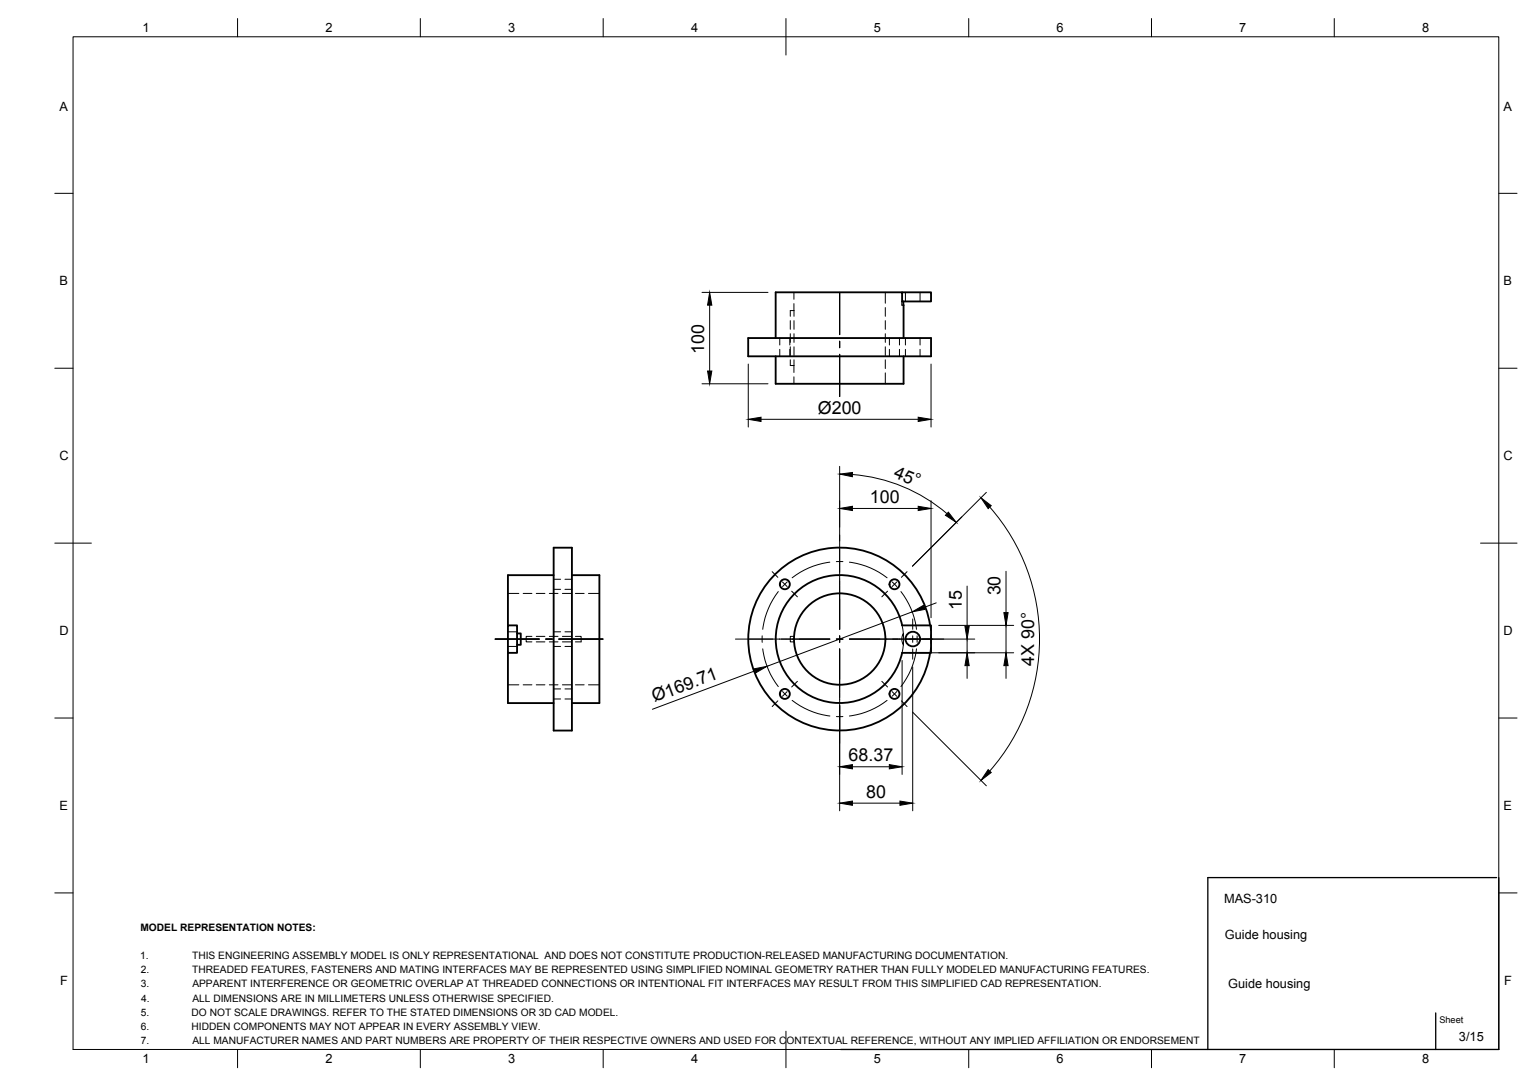
ISO-10303-21;
HEADER;
/* Generated by software containing ST-Developer
 * from STEP Tools, Inc. (www.steptools.com) 
 */

FILE_DESCRIPTION(
/* description */ ('Independent30mm screw-fed quill/spindle unit with16mm straight tool s
ocket, radial set screw, native reusable open ball bearings, retained 
inner/outer race stacks, keyed quill guide and M12x1.75 fine feed. Ext
ernal moving drive and tool not included. Ideal cage orbital links; in
dividual ball spin, force and preload not simulated. No drilling capac
ity, runout, speed, torque, load, life or machine safety rating.'),
/* implementation_level */ '2;1');

FILE_NAME(
/* name */ 'Guide housing.step',
/* time_stamp */ '2026-11-08T18:59:42-08:00',
/* author */ (''),
/* organization */ (''),
/* preprocessor_version */ 'ST-DEVELOPER v20.2',
/* originating_system */ 'Autodesk Translation Framework v15.17.0.0',
/* authorisation */ '');

FILE_SCHEMA (('AUTOMOTIVE_DESIGN { 1 0 10303 214 3 1 1 }'));
ENDSEC;

DATA;
#10=MECHANICAL_DESIGN_GEOMETRIC_PRESENTATION_REPRESENTATION('',(#1592),#63898);
#1556=SHAPE_REPRESENTATION_RELATIONSHIP('SRR','None',#63995,#1574);
#1574=ADVANCED_BREP_SHAPE_REPRESENTATION('',(#1610),#63880);
#1592=STYLED_ITEM('',(#64094),#1610);
#1610=MANIFOLD_SOLID_BREP('Body1',#15478);
#1628=FACE_BOUND('',#3516,.T.);
#1629=FACE_BOUND('',#3518,.T.);
#1630=FACE_BOUND('',#3519,.T.);
#1631=FACE_BOUND('',#3520,.T.);
#1632=FACE_BOUND('',#3521,.T.);
#1633=FACE_BOUND('',#3522,.T.);
#1634=FACE_BOUND('',#3523,.T.);
#1635=FACE_BOUND('',#3525,.T.);
#1636=FACE_BOUND('',#3526,.T.);
#1637=FACE_BOUND('',#3527,.T.);
#1638=FACE_BOUND('',#3528,.T.);
#1639=FACE_BOUND('',#3529,.T.);
#1640=FACE_BOUND('',#3530,.T.);
#1641=FACE_BOUND('',#3535,.T.);
#1642=FACE_BOUND('',#3536,.T.);
#1643=FACE_BOUND('',#3538,.T.);
#1715=CYLINDRICAL_SURFACE('',#15709,12.);
#1716=CYLINDRICAL_SURFACE('',#15711,70.);
#1717=CYLINDRICAL_SURFACE('',#15717,8.);
#1718=CYLINDRICAL_SURFACE('',#15720,8.);
#1719=CYLINDRICAL_SURFACE('',#15723,5.5);
#1720=CYLINDRICAL_SURFACE('',#15726,5.5);
#1721=CYLINDRICAL_SURFACE('',#15729,5.5);
#1722=CYLINDRICAL_SURFACE('',#15732,5.5);
#1723=CYLINDRICAL_SURFACE('',#15744,100.);
#1724=CYLINDRICAL_SURFACE('',#15745,70.);
#1725=CYLINDRICAL_SURFACE('',#15747,50.);
#2380=CIRCLE('',#15699,50.);
#2381=CIRCLE('',#15700,50.);
#2382=CIRCLE('',#15704,50.);
#2383=CIRCLE('',#15705,50.);
#2384=CIRCLE('',#15707,70.);
#2385=CIRCLE('',#15708,12.);
#2386=CIRCLE('',#15710,12.);
#2387=CIRCLE('',#15712,70.);
#2388=CIRCLE('',#15713,70.);
#2389=CIRCLE('',#15714,70.);
#2390=CIRCLE('',#15715,70.);
#2391=CIRCLE('',#15716,70.);
#2392=CIRCLE('',#15718,8.);
#2393=CIRCLE('',#15719,8.);
#2394=CIRCLE('',#15721,8.);
#2395=CIRCLE('',#15722,8.);
#2396=CIRCLE('',#15724,5.5);
#2397=CIRCLE('',#15725,5.5);
#2398=CIRCLE('',#15727,5.5);
#2399=CIRCLE('',#15728,5.5);
#2400=CIRCLE('',#15730,5.5);
#2401=CIRCLE('',#15731,5.5);
#2402=CIRCLE('',#15733,5.5);
#2403=CIRCLE('',#15734,5.5);
#2404=CIRCLE('',#15740,100.);
#2405=CIRCLE('',#15742,100.);
#2406=CIRCLE('',#15743,70.);
#2407=CIRCLE('',#15746,70.);
#2408=CIRCLE('',#15748,50.);
#2409=CIRCLE('',#15749,50.);
#2660=FACE_OUTER_BOUND('',#3498,.T.);
#2661=FACE_OUTER_BOUND('',#3499,.T.);
#2662=FACE_OUTER_BOUND('',#3500,.T.);
#2663=FACE_OUTER_BOUND('',#3501,.T.);
#2664=FACE_OUTER_BOUND('',#3502,.T.);
#2665=FACE_OUTER_BOUND('',#3503,.T.);
#2666=FACE_OUTER_BOUND('',#3504,.T.);
#2667=FACE_OUTER_BOUND('',#3505,.T.);
#2668=FACE_OUTER_BOUND('',#3506,.T.);
#2669=FACE_OUTER_BOUND('',#3507,.T.);
#2670=FACE_OUTER_BOUND('',#3508,.T.);
#2671=FACE_OUTER_BOUND('',#3509,.T.);
#2672=FACE_OUTER_BOUND('',#3510,.T.);
#2673=FACE_OUTER_BOUND('',#3511,.T.);
#2674=FACE_OUTER_BOUND('',#3512,.T.);
#2675=FACE_OUTER_BOUND('',#3513,.T.);
#2676=FACE_OUTER_BOUND('',#3514,.T.);
#2677=FACE_OUTER_BOUND('',#3515,.T.);
#2678=FACE_OUTER_BOUND('',#3517,.T.);
#2679=FACE_OUTER_BOUND('',#3524,.T.);
#2680=FACE_OUTER_BOUND('',#3531,.T.);
#2681=FACE_OUTER_BOUND('',#3532,.T.);
#2682=FACE_OUTER_BOUND('',#3533,.T.);
#2683=FACE_OUTER_BOUND('',#3534,.T.);
#2684=FACE_OUTER_BOUND('',#3537,.T.);
#3498=EDGE_LOOP('',(#9844,#9845,#9846,#9847));
#3499=EDGE_LOOP('',(#9848,#9849,#9850,#9851,#9852));
#3500=EDGE_LOOP('',(#9853,#9854,#9855,#9856));
#3501=EDGE_LOOP('',(#9857,#9858,#9859,#9860));
#3502=EDGE_LOOP('',(#9861,#9862,#9863,#9864,#9865));
#3503=EDGE_LOOP('',(#9866,#9867));
#3504=EDGE_LOOP('',(#9868,#9869,#9870,#9871));
#3505=EDGE_LOOP('',(#9872,#9873,#9874,#9875,#9876,#9877,#9878,#9879,#9880,
#9881,#9882,#9883));
#3506=EDGE_LOOP('',(#9884,#9885,#9886,#9887));
#3507=EDGE_LOOP('',(#9888,#9889,#9890,#9891));
#3508=EDGE_LOOP('',(#9892,#9893,#9894,#9895));
#3509=EDGE_LOOP('',(#9896,#9897,#9898,#9899));
#3510=EDGE_LOOP('',(#9900,#9901,#9902,#9903));
#3511=EDGE_LOOP('',(#9904,#9905,#9906,#9907));
#3512=EDGE_LOOP('',(#9908,#9909,#9910,#9911));
#3513=EDGE_LOOP('',(#9912,#9913,#9914,#9915));
#3514=EDGE_LOOP('',(#9916,#9917,#9918,#9919));
#3515=EDGE_LOOP('',(#9920,#9921,#9922,#9923,#9924,#9925));
#3516=EDGE_LOOP('',(#9926));
#3517=EDGE_LOOP('',(#9927));
#3518=EDGE_LOOP('',(#9928));
#3519=EDGE_LOOP('',(#9929));
#3520=EDGE_LOOP('',(#9930));
#3521=EDGE_LOOP('',(#9931));
#3522=EDGE_LOOP('',(#9932));
#3523=EDGE_LOOP('',(#9933));
#3524=EDGE_LOOP('',(#9934));
#3525=EDGE_LOOP('',(#9935));
#3526=EDGE_LOOP('',(#9936));
#3527=EDGE_LOOP('',(#9937));
#3528=EDGE_LOOP('',(#9938));
#3529=EDGE_LOOP('',(#9939));
#3530=EDGE_LOOP('',(#9940));
#3531=EDGE_LOOP('',(#9941,#9942,#9943,#9944));
#3532=EDGE_LOOP('',(#9945,#9946,#9947,#9948));
#3533=EDGE_LOOP('',(#9949,#9950,#9951,#9952,#9953,#9954,#9955,#9956,#9957,
#9958,#9959,#9960));
#3534=EDGE_LOOP('',(#9961,#9962,#9963,#9964,#9965));
#3535=EDGE_LOOP('',(#9966));
#3536=EDGE_LOOP('',(#9967));
#3537=EDGE_LOOP('',(#9968));
#3538=EDGE_LOOP('',(#9969));
#4423=LINE('',#19955,#5186);
#4424=LINE('',#19957,#5187);
#4425=LINE('',#19959,#5188);
#4426=LINE('',#19960,#5189);
#4427=LINE('',#19965,#5190);
#4428=LINE('',#19967,#5191);
#4429=LINE('',#19971,#5192);
#4430=LINE('',#19973,#5193);
#4431=LINE('',#19974,#5194);
#4432=LINE('',#19976,#5195);
#4433=LINE('',#19988,#5196);
#4434=LINE('',#19991,#5197);
#4435=LINE('',#19996,#5198);
#4436=LINE('',#20000,#5199);
#4437=LINE('',#20005,#5200);
#4438=LINE('',#20011,#5201);
#4439=LINE('',#20017,#5202);
#4440=LINE('',#20023,#5203);
#4441=LINE('',#20029,#5204);
#4442=LINE('',#20035,#5205);
#4443=LINE('',#20041,#5206);
#4444=LINE('',#20045,#5207);
#4445=LINE('',#20047,#5208);
#4446=LINE('',#20048,#5209);
#4447=LINE('',#20051,#5210);
#4448=LINE('',#20053,#5211);
#4449=LINE('',#20054,#5212);
#4450=LINE('',#20056,#5213);
#4451=LINE('',#20057,#5214);
#4452=LINE('',#20068,#5215);
#4453=LINE('',#20071,#5216);
#4454=LINE('',#20076,#5217);
#4455=LINE('',#20078,#5218);
#5186=VECTOR('',#16865,10.);
#5187=VECTOR('',#16866,10.);
#5188=VECTOR('',#16867,10.);
#5189=VECTOR('',#16868,10.);
#5190=VECTOR('',#16873,10.);
#5191=VECTOR('',#16874,10.);
#5192=VECTOR('',#16879,10.);
#5193=VECTOR('',#16880,10.);
#5194=VECTOR('',#16881,10.);
#5195=VECTOR('',#16884,10.);
#5196=VECTOR('',#16899,10.);
#5197=VECTOR('',#16902,10.);
#5198=VECTOR('',#16907,10.);
#5199=VECTOR('',#16910,70.);
#5200=VECTOR('',#16915,10.);
#5201=VECTOR('',#16922,8.);
#5202=VECTOR('',#16929,8.);
#5203=VECTOR('',#16936,5.5);
#5204=VECTOR('',#16943,5.5);
#5205=VECTOR('',#16950,5.5);
#5206=VECTOR('',#16957,5.5);
#5207=VECTOR('',#16962,10.);
#5208=VECTOR('',#16963,10.);
#5209=VECTOR('',#16964,10.);
#5210=VECTOR('',#16967,10.);
#5211=VECTOR('',#16968,10.);
#5212=VECTOR('',#16969,10.);
#5213=VECTOR('',#16972,10.);
#5214=VECTOR('',#16973,10.);
#5215=VECTOR('',#16988,100.);
#5216=VECTOR('',#16991,70.);
#5217=VECTOR('',#16998,50.);
#5218=VECTOR('',#16999,50.);
#5949=VERTEX_POINT('',#19953);
#5950=VERTEX_POINT('',#19954);
#5951=VERTEX_POINT('',#19956);
#5952=VERTEX_POINT('',#19958);
#5953=VERTEX_POINT('',#19962);
#5954=VERTEX_POINT('',#19964);
#5955=VERTEX_POINT('',#19966);
#5956=VERTEX_POINT('',#19970);
#5957=VERTEX_POINT('',#19972);
#5958=VERTEX_POINT('',#19978);
#5959=VERTEX_POINT('',#19982);
#5960=VERTEX_POINT('',#19983);
#5961=VERTEX_POINT('',#19987);
#5962=VERTEX_POINT('',#19989);
#5963=VERTEX_POINT('',#19993);
#5964=VERTEX_POINT('',#19995);
#5965=VERTEX_POINT('',#19997);
#5966=VERTEX_POINT('',#19999);
#5967=VERTEX_POINT('',#20002);
#5968=VERTEX_POINT('',#20004);
#5969=VERTEX_POINT('',#20008);
#5970=VERTEX_POINT('',#20010);
#5971=VERTEX_POINT('',#20014);
#5972=VERTEX_POINT('',#20016);
#5973=VERTEX_POINT('',#20020);
#5974=VERTEX_POINT('',#20022);
#5975=VERTEX_POINT('',#20026);
#5976=VERTEX_POINT('',#20028);
#5977=VERTEX_POINT('',#20032);
#5978=VERTEX_POINT('',#20034);
#5979=VERTEX_POINT('',#20038);
#5980=VERTEX_POINT('',#20040);
#5981=VERTEX_POINT('',#20044);
#5982=VERTEX_POINT('',#20046);
#5983=VERTEX_POINT('',#20050);
#5984=VERTEX_POINT('',#20052);
#5985=VERTEX_POINT('',#20060);
#5986=VERTEX_POINT('',#20063);
#5987=VERTEX_POINT('',#20065);
#5988=VERTEX_POINT('',#20070);
#5989=VERTEX_POINT('',#20074);
#5990=VERTEX_POINT('',#20077);
#7511=EDGE_CURVE('',#5949,#5950,#4423,.T.);
#7512=EDGE_CURVE('',#5949,#5951,#4424,.T.);
#7513=EDGE_CURVE('',#5952,#5951,#4425,.T.);
#7514=EDGE_CURVE('',#5952,#5950,#4426,.T.);
#7515=EDGE_CURVE('',#5950,#5953,#2380,.T.);
#7516=EDGE_CURVE('',#5954,#5952,#4427,.T.);
#7517=EDGE_CURVE('',#5955,#5954,#4428,.T.);
#7518=EDGE_CURVE('',#5953,#5955,#2381,.T.);
#7519=EDGE_CURVE('',#5955,#5956,#4429,.T.);
#7520=EDGE_CURVE('',#5954,#5957,#4430,.T.);
#7521=EDGE_CURVE('',#5957,#5956,#4431,.T.);
#7522=EDGE_CURVE('',#5951,#5957,#4432,.T.);
#7523=EDGE_CURVE('',#5956,#5958,#2382,.T.);
#7524=EDGE_CURVE('',#5958,#5949,#2383,.T.);
#7525=EDGE_CURVE('',#5959,#5960,#2384,.T.);
#7526=EDGE_CURVE('',#5960,#5959,#2385,.T.);
#7527=EDGE_CURVE('',#5961,#5959,#4433,.T.);
#7528=EDGE_CURVE('',#5961,#5962,#2386,.T.);
#7529=EDGE_CURVE('',#5960,#5962,#4434,.T.);
#7530=EDGE_CURVE('',#5962,#5963,#2387,.T.);
#7531=EDGE_CURVE('',#5963,#5964,#4435,.T.);
#7532=EDGE_CURVE('',#5965,#5964,#2388,.T.);
#7533=EDGE_CURVE('',#5965,#5966,#4436,.T.);
#7534=EDGE_CURVE('',#5966,#5966,#2389,.T.);
#7535=EDGE_CURVE('',#5967,#5965,#2390,.T.);
#7536=EDGE_CURVE('',#5967,#5968,#4437,.T.);
#7537=EDGE_CURVE('',#5968,#5961,#2391,.T.);
#7538=EDGE_CURVE('',#5969,#5969,#2392,.T.);
#7539=EDGE_CURVE('',#5969,#5970,#4438,.T.);
#7540=EDGE_CURVE('',#5970,#5970,#2393,.T.);
#7541=EDGE_CURVE('',#5971,#5971,#2394,.T.);
#7542=EDGE_CURVE('',#5971,#5972,#4439,.T.);
#7543=EDGE_CURVE('',#5972,#5972,#2395,.T.);
#7544=EDGE_CURVE('',#5973,#5973,#2396,.T.);
#7545=EDGE_CURVE('',#5973,#5974,#4440,.T.);
#7546=EDGE_CURVE('',#5974,#5974,#2397,.T.);
#7547=EDGE_CURVE('',#5975,#5975,#2398,.T.);
#7548=EDGE_CURVE('',#5975,#5976,#4441,.T.);
#7549=EDGE_CURVE('',#5976,#5976,#2399,.T.);
#7550=EDGE_CURVE('',#5977,#5977,#2400,.T.);
#7551=EDGE_CURVE('',#5977,#5978,#4442,.T.);
#7552=EDGE_CURVE('',#5978,#5978,#2401,.T.);
#7553=EDGE_CURVE('',#5979,#5979,#2402,.T.);
#7554=EDGE_CURVE('',#5979,#5980,#4443,.T.);
#7555=EDGE_CURVE('',#5980,#5980,#2403,.T.);
#7556=EDGE_CURVE('',#5981,#5967,#4444,.T.);
#7557=EDGE_CURVE('',#5982,#5981,#4445,.T.);
#7558=EDGE_CURVE('',#5982,#5968,#4446,.T.);
#7559=EDGE_CURVE('',#5983,#5982,#4447,.T.);
#7560=EDGE_CURVE('',#5984,#5981,#4448,.T.);
#7561=EDGE_CURVE('',#5983,#5984,#4449,.T.);
#7562=EDGE_CURVE('',#5963,#5983,#4450,.T.);
#7563=EDGE_CURVE('',#5964,#5984,#4451,.T.);
#7564=EDGE_CURVE('',#5985,#5985,#2404,.T.);
#7565=EDGE_CURVE('',#5986,#5986,#2405,.T.);
#7566=EDGE_CURVE('',#5987,#5987,#2406,.T.);
#7567=EDGE_CURVE('',#5985,#5986,#4452,.T.);
#7568=EDGE_CURVE('',#5987,#5988,#4453,.T.);
#7569=EDGE_CURVE('',#5988,#5988,#2407,.T.);
#7570=EDGE_CURVE('',#5989,#5989,#2408,.T.);
#7571=EDGE_CURVE('',#5989,#5953,#4454,.T.);
#7572=EDGE_CURVE('',#5958,#5990,#4455,.T.);
#7573=EDGE_CURVE('',#5990,#5990,#2409,.T.);
#9844=ORIENTED_EDGE('',*,*,#7511,.F.);
#9845=ORIENTED_EDGE('',*,*,#7512,.T.);
#9846=ORIENTED_EDGE('',*,*,#7513,.F.);
#9847=ORIENTED_EDGE('',*,*,#7514,.T.);
#9848=ORIENTED_EDGE('',*,*,#7515,.F.);
#9849=ORIENTED_EDGE('',*,*,#7514,.F.);
#9850=ORIENTED_EDGE('',*,*,#7516,.F.);
#9851=ORIENTED_EDGE('',*,*,#7517,.F.);
#9852=ORIENTED_EDGE('',*,*,#7518,.F.);
#9853=ORIENTED_EDGE('',*,*,#7519,.F.);
#9854=ORIENTED_EDGE('',*,*,#7517,.T.);
#9855=ORIENTED_EDGE('',*,*,#7520,.T.);
#9856=ORIENTED_EDGE('',*,*,#7521,.T.);
#9857=ORIENTED_EDGE('',*,*,#7516,.T.);
#9858=ORIENTED_EDGE('',*,*,#7513,.T.);
#9859=ORIENTED_EDGE('',*,*,#7522,.T.);
#9860=ORIENTED_EDGE('',*,*,#7520,.F.);
#9861=ORIENTED_EDGE('',*,*,#7523,.F.);
#9862=ORIENTED_EDGE('',*,*,#7521,.F.);
#9863=ORIENTED_EDGE('',*,*,#7522,.F.);
#9864=ORIENTED_EDGE('',*,*,#7512,.F.);
#9865=ORIENTED_EDGE('',*,*,#7524,.F.);
#9866=ORIENTED_EDGE('',*,*,#7525,.F.);
#9867=ORIENTED_EDGE('',*,*,#7526,.F.);
#9868=ORIENTED_EDGE('',*,*,#7527,.F.);
#9869=ORIENTED_EDGE('',*,*,#7528,.T.);
#9870=ORIENTED_EDGE('',*,*,#7529,.F.);
#9871=ORIENTED_EDGE('',*,*,#7526,.T.);
#9872=ORIENTED_EDGE('',*,*,#7527,.T.);
#9873=ORIENTED_EDGE('',*,*,#7525,.T.);
#9874=ORIENTED_EDGE('',*,*,#7529,.T.);
#9875=ORIENTED_EDGE('',*,*,#7530,.T.);
#9876=ORIENTED_EDGE('',*,*,#7531,.T.);
#9877=ORIENTED_EDGE('',*,*,#7532,.F.);
#9878=ORIENTED_EDGE('',*,*,#7533,.T.);
#9879=ORIENTED_EDGE('',*,*,#7534,.T.);
#9880=ORIENTED_EDGE('',*,*,#7533,.F.);
#9881=ORIENTED_EDGE('',*,*,#7535,.F.);
#9882=ORIENTED_EDGE('',*,*,#7536,.T.);
#9883=ORIENTED_EDGE('',*,*,#7537,.T.);
#9884=ORIENTED_EDGE('',*,*,#7538,.F.);
#9885=ORIENTED_EDGE('',*,*,#7539,.T.);
#9886=ORIENTED_EDGE('',*,*,#7540,.F.);
#9887=ORIENTED_EDGE('',*,*,#7539,.F.);
#9888=ORIENTED_EDGE('',*,*,#7541,.F.);
#9889=ORIENTED_EDGE('',*,*,#7542,.T.);
#9890=ORIENTED_EDGE('',*,*,#7543,.F.);
#9891=ORIENTED_EDGE('',*,*,#7542,.F.);
#9892=ORIENTED_EDGE('',*,*,#7544,.F.);
#9893=ORIENTED_EDGE('',*,*,#7545,.T.);
#9894=ORIENTED_EDGE('',*,*,#7546,.F.);
#9895=ORIENTED_EDGE('',*,*,#7545,.F.);
#9896=ORIENTED_EDGE('',*,*,#7547,.F.);
#9897=ORIENTED_EDGE('',*,*,#7548,.T.);
#9898=ORIENTED_EDGE('',*,*,#7549,.F.);
#9899=ORIENTED_EDGE('',*,*,#7548,.F.);
#9900=ORIENTED_EDGE('',*,*,#7550,.F.);
#9901=ORIENTED_EDGE('',*,*,#7551,.T.);
#9902=ORIENTED_EDGE('',*,*,#7552,.F.);
#9903=ORIENTED_EDGE('',*,*,#7551,.F.);
#9904=ORIENTED_EDGE('',*,*,#7553,.F.);
#9905=ORIENTED_EDGE('',*,*,#7554,.T.);
#9906=ORIENTED_EDGE('',*,*,#7555,.F.);
#9907=ORIENTED_EDGE('',*,*,#7554,.F.);
#9908=ORIENTED_EDGE('',*,*,#7536,.F.);
#9909=ORIENTED_EDGE('',*,*,#7556,.F.);
#9910=ORIENTED_EDGE('',*,*,#7557,.F.);
#9911=ORIENTED_EDGE('',*,*,#7558,.T.);
#9912=ORIENTED_EDGE('',*,*,#7559,.T.);
#9913=ORIENTED_EDGE('',*,*,#7557,.T.);
#9914=ORIENTED_EDGE('',*,*,#7560,.F.);
#9915=ORIENTED_EDGE('',*,*,#7561,.F.);
#9916=ORIENTED_EDGE('',*,*,#7531,.F.);
#9917=ORIENTED_EDGE('',*,*,#7562,.T.);
#9918=ORIENTED_EDGE('',*,*,#7561,.T.);
#9919=ORIENTED_EDGE('',*,*,#7563,.F.);
#9920=ORIENTED_EDGE('',*,*,#7537,.F.);
#9921=ORIENTED_EDGE('',*,*,#7558,.F.);
#9922=ORIENTED_EDGE('',*,*,#7559,.F.);
#9923=ORIENTED_EDGE('',*,*,#7562,.F.);
#9924=ORIENTED_EDGE('',*,*,#7530,.F.);
#9925=ORIENTED_EDGE('',*,*,#7528,.F.);
#9926=ORIENTED_EDGE('',*,*,#7540,.T.);
#9927=ORIENTED_EDGE('',*,*,#7564,.T.);
#9928=ORIENTED_EDGE('',*,*,#7541,.T.);
#9929=ORIENTED_EDGE('',*,*,#7534,.F.);
#9930=ORIENTED_EDGE('',*,*,#7553,.T.);
#9931=ORIENTED_EDGE('',*,*,#7550,.T.);
#9932=ORIENTED_EDGE('',*,*,#7547,.T.);
#9933=ORIENTED_EDGE('',*,*,#7544,.T.);
#9934=ORIENTED_EDGE('',*,*,#7565,.F.);
#9935=ORIENTED_EDGE('',*,*,#7543,.T.);
#9936=ORIENTED_EDGE('',*,*,#7566,.F.);
#9937=ORIENTED_EDGE('',*,*,#7555,.T.);
#9938=ORIENTED_EDGE('',*,*,#7552,.T.);
#9939=ORIENTED_EDGE('',*,*,#7549,.T.);
#9940=ORIENTED_EDGE('',*,*,#7546,.T.);
#9941=ORIENTED_EDGE('',*,*,#7564,.F.);
#9942=ORIENTED_EDGE('',*,*,#7567,.T.);
#9943=ORIENTED_EDGE('',*,*,#7565,.T.);
#9944=ORIENTED_EDGE('',*,*,#7567,.F.);
#9945=ORIENTED_EDGE('',*,*,#7566,.T.);
#9946=ORIENTED_EDGE('',*,*,#7568,.T.);
#9947=ORIENTED_EDGE('',*,*,#7569,.T.);
#9948=ORIENTED_EDGE('',*,*,#7568,.F.);
#9949=ORIENTED_EDGE('',*,*,#7570,.F.);
#9950=ORIENTED_EDGE('',*,*,#7571,.T.);
#9951=ORIENTED_EDGE('',*,*,#7518,.T.);
#9952=ORIENTED_EDGE('',*,*,#7519,.T.);
#9953=ORIENTED_EDGE('',*,*,#7523,.T.);
#9954=ORIENTED_EDGE('',*,*,#7572,.T.);
#9955=ORIENTED_EDGE('',*,*,#7573,.T.);
#9956=ORIENTED_EDGE('',*,*,#7572,.F.);
#9957=ORIENTED_EDGE('',*,*,#7524,.T.);
#9958=ORIENTED_EDGE('',*,*,#7511,.T.);
#9959=ORIENTED_EDGE('',*,*,#7515,.T.);
#9960=ORIENTED_EDGE('',*,*,#7571,.F.);
#9961=ORIENTED_EDGE('',*,*,#7535,.T.);
#9962=ORIENTED_EDGE('',*,*,#7532,.T.);
#9963=ORIENTED_EDGE('',*,*,#7563,.T.);
#9964=ORIENTED_EDGE('',*,*,#7560,.T.);
#9965=ORIENTED_EDGE('',*,*,#7556,.T.);
#9966=ORIENTED_EDGE('',*,*,#7538,.T.);
#9967=ORIENTED_EDGE('',*,*,#7570,.T.);
#9968=ORIENTED_EDGE('',*,*,#7569,.F.);
#9969=ORIENTED_EDGE('',*,*,#7573,.F.);
#14510=PLANE('',#15697);
#14511=PLANE('',#15698);
#14512=PLANE('',#15701);
#14513=PLANE('',#15702);
#14514=PLANE('',#15703);
#14515=PLANE('',#15706);
#14516=PLANE('',#15735);
#14517=PLANE('',#15736);
#14518=PLANE('',#15737);
#14519=PLANE('',#15738);
#14520=PLANE('',#15739);
#14521=PLANE('',#15741);
#14522=PLANE('',#15750);
#14523=PLANE('',#15751);
#14640=ADVANCED_FACE('',(#2660),#14510,.F.);
#14641=ADVANCED_FACE('',(#2661),#14511,.F.);
#14642=ADVANCED_FACE('',(#2662),#14512,.F.);
#14643=ADVANCED_FACE('',(#2663),#14513,.F.);
#14644=ADVANCED_FACE('',(#2664),#14514,.F.);
#14645=ADVANCED_FACE('',(#2665),#14515,.F.);
#14646=ADVANCED_FACE('',(#2666),#1715,.F.);
#14647=ADVANCED_FACE('',(#2667),#1716,.T.);
#14648=ADVANCED_FACE('',(#2668),#1717,.F.);
#14649=ADVANCED_FACE('',(#2669),#1718,.F.);
#14650=ADVANCED_FACE('',(#2670),#1719,.F.);
#14651=ADVANCED_FACE('',(#2671),#1720,.F.);
#14652=ADVANCED_FACE('',(#2672),#1721,.F.);
#14653=ADVANCED_FACE('',(#2673),#1722,.F.);
#14654=ADVANCED_FACE('',(#2674),#14516,.T.);
#14655=ADVANCED_FACE('',(#2675),#14517,.T.);
#14656=ADVANCED_FACE('',(#2676),#14518,.T.);
#14657=ADVANCED_FACE('',(#2677,#1628),#14519,.F.);
#14658=ADVANCED_FACE('',(#2678,#1629,#1630,#1631,#1632,#1633,#1634),#14520,
 .T.);
#14659=ADVANCED_FACE('',(#2679,#1635,#1636,#1637,#1638,#1639,#1640),#14521,
 .F.);
#14660=ADVANCED_FACE('',(#2680),#1723,.T.);
#14661=ADVANCED_FACE('',(#2681),#1724,.T.);
#14662=ADVANCED_FACE('',(#2682),#1725,.F.);
#14663=ADVANCED_FACE('',(#2683,#1641,#1642),#14522,.T.);
#14664=ADVANCED_FACE('',(#2684,#1643),#14523,.F.);
#15478=CLOSED_SHELL('',(#14640,#14641,#14642,#14643,#14644,#14645,#14646,
#14647,#14648,#14649,#14650,#14651,#14652,#14653,#14654,#14655,#14656,#14657,
#14658,#14659,#14660,#14661,#14662,#14663,#14664));
#15696=AXIS2_PLACEMENT_3D('',#19951,#16861,#16862);
#15697=AXIS2_PLACEMENT_3D('',#19952,#16863,#16864);
#15698=AXIS2_PLACEMENT_3D('',#19961,#16869,#16870);
#15699=AXIS2_PLACEMENT_3D('',#19963,#16871,#16872);
#15700=AXIS2_PLACEMENT_3D('',#19968,#16875,#16876);
#15701=AXIS2_PLACEMENT_3D('',#19969,#16877,#16878);
#15702=AXIS2_PLACEMENT_3D('',#19975,#16882,#16883);
#15703=AXIS2_PLACEMENT_3D('',#19977,#16885,#16886);
#15704=AXIS2_PLACEMENT_3D('',#19979,#16887,#16888);
#15705=AXIS2_PLACEMENT_3D('',#19980,#16889,#16890);
#15706=AXIS2_PLACEMENT_3D('',#19981,#16891,#16892);
#15707=AXIS2_PLACEMENT_3D('',#19984,#16893,#16894);
#15708=AXIS2_PLACEMENT_3D('',#19985,#16895,#16896);
#15709=AXIS2_PLACEMENT_3D('',#19986,#16897,#16898);
#15710=AXIS2_PLACEMENT_3D('',#19990,#16900,#16901);
#15711=AXIS2_PLACEMENT_3D('',#19992,#16903,#16904);
#15712=AXIS2_PLACEMENT_3D('',#19994,#16905,#16906);
#15713=AXIS2_PLACEMENT_3D('',#19998,#16908,#16909);
#15714=AXIS2_PLACEMENT_3D('',#20001,#16911,#16912);
#15715=AXIS2_PLACEMENT_3D('',#20003,#16913,#16914);
#15716=AXIS2_PLACEMENT_3D('',#20006,#16916,#16917);
#15717=AXIS2_PLACEMENT_3D('',#20007,#16918,#16919);
#15718=AXIS2_PLACEMENT_3D('',#20009,#16920,#16921);
#15719=AXIS2_PLACEMENT_3D('',#20012,#16923,#16924);
#15720=AXIS2_PLACEMENT_3D('',#20013,#16925,#16926);
#15721=AXIS2_PLACEMENT_3D('',#20015,#16927,#16928);
#15722=AXIS2_PLACEMENT_3D('',#20018,#16930,#16931);
#15723=AXIS2_PLACEMENT_3D('',#20019,#16932,#16933);
#15724=AXIS2_PLACEMENT_3D('',#20021,#16934,#16935);
#15725=AXIS2_PLACEMENT_3D('',#20024,#16937,#16938);
#15726=AXIS2_PLACEMENT_3D('',#20025,#16939,#16940);
#15727=AXIS2_PLACEMENT_3D('',#20027,#16941,#16942);
#15728=AXIS2_PLACEMENT_3D('',#20030,#16944,#16945);
#15729=AXIS2_PLACEMENT_3D('',#20031,#16946,#16947);
#15730=AXIS2_PLACEMENT_3D('',#20033,#16948,#16949);
#15731=AXIS2_PLACEMENT_3D('',#20036,#16951,#16952);
#15732=AXIS2_PLACEMENT_3D('',#20037,#16953,#16954);
#15733=AXIS2_PLACEMENT_3D('',#20039,#16955,#16956);
#15734=AXIS2_PLACEMENT_3D('',#20042,#16958,#16959);
#15735=AXIS2_PLACEMENT_3D('',#20043,#16960,#16961);
#15736=AXIS2_PLACEMENT_3D('',#20049,#16965,#16966);
#15737=AXIS2_PLACEMENT_3D('',#20055,#16970,#16971);
#15738=AXIS2_PLACEMENT_3D('',#20058,#16974,#16975);
#15739=AXIS2_PLACEMENT_3D('',#20059,#16976,#16977);
#15740=AXIS2_PLACEMENT_3D('',#20061,#16978,#16979);
#15741=AXIS2_PLACEMENT_3D('',#20062,#16980,#16981);
#15742=AXIS2_PLACEMENT_3D('',#20064,#16982,#16983);
#15743=AXIS2_PLACEMENT_3D('',#20066,#16984,#16985);
#15744=AXIS2_PLACEMENT_3D('',#20067,#16986,#16987);
#15745=AXIS2_PLACEMENT_3D('',#20069,#16989,#16990);
#15746=AXIS2_PLACEMENT_3D('',#20072,#16992,#16993);
#15747=AXIS2_PLACEMENT_3D('',#20073,#16994,#16995);
#15748=AXIS2_PLACEMENT_3D('',#20075,#16996,#16997);
#15749=AXIS2_PLACEMENT_3D('',#20079,#17000,#17001);
#15750=AXIS2_PLACEMENT_3D('',#20080,#17002,#17003);
#15751=AXIS2_PLACEMENT_3D('',#20081,#17004,#17005);
#16861=DIRECTION('axis',(0.,0.,1.));
#16862=DIRECTION('refdir',(1.,0.,0.));
#16863=DIRECTION('center_axis',(0.,-1.,0.));
#16864=DIRECTION('ref_axis',(-1.,0.,0.));
#16865=DIRECTION('',(0.,0.,1.));
#16866=DIRECTION('',(-1.,0.,0.));
#16867=DIRECTION('',(0.,0.,-1.));
#16868=DIRECTION('',(1.,0.,0.));
#16869=DIRECTION('center_axis',(0.,0.,1.));
#16870=DIRECTION('ref_axis',(1.,0.,0.));
#16871=DIRECTION('center_axis',(0.,0.,-1.));
#16872=DIRECTION('ref_axis',(1.,0.,0.));
#16873=DIRECTION('',(0.,-1.,0.));
#16874=DIRECTION('',(-1.,0.,0.));
#16875=DIRECTION('center_axis',(0.,0.,-1.));
#16876=DIRECTION('ref_axis',(1.,0.,0.));
#16877=DIRECTION('center_axis',(0.,1.,0.));
#16878=DIRECTION('ref_axis',(1.,0.,0.));
#16879=DIRECTION('',(0.,0.,-1.));
#16880=DIRECTION('',(0.,0.,-1.));
#16881=DIRECTION('',(1.,0.,0.));
#16882=DIRECTION('center_axis',(-1.,0.,0.));
#16883=DIRECTION('ref_axis',(0.,1.,0.));
#16884=DIRECTION('',(0.,1.,0.));
#16885=DIRECTION('center_axis',(0.,0.,-1.));
#16886=DIRECTION('ref_axis',(-1.,0.,0.));
#16887=DIRECTION('center_axis',(0.,0.,1.));
#16888=DIRECTION('ref_axis',(1.,0.,0.));
#16889=DIRECTION('center_axis',(0.,0.,1.));
#16890=DIRECTION('ref_axis',(1.,0.,0.));
#16891=DIRECTION('center_axis',(0.,0.,-1.));
#16892=DIRECTION('ref_axis',(1.,0.,0.));
#16893=DIRECTION('center_axis',(0.,0.,-1.));
#16894=DIRECTION('ref_axis',(1.,0.,0.));
#16895=DIRECTION('center_axis',(0.,0.,-1.));
#16896=DIRECTION('ref_axis',(1.,0.,0.));
#16897=DIRECTION('center_axis',(0.,0.,-1.));
#16898=DIRECTION('ref_axis',(-1.,1.22464679914735E-16,0.));
#16899=DIRECTION('',(0.,0.,-1.));
#16900=DIRECTION('center_axis',(0.,0.,1.));
#16901=DIRECTION('ref_axis',(1.,0.,0.));
#16902=DIRECTION('',(0.,0.,1.));
#16903=DIRECTION('center_axis',(0.,0.,1.));
#16904=DIRECTION('ref_axis',(1.,0.,0.));
#16905=DIRECTION('center_axis',(0.,0.,-1.));
#16906=DIRECTION('ref_axis',(1.,0.,0.));
#16907=DIRECTION('',(0.,0.,1.));
#16908=DIRECTION('center_axis',(0.,0.,1.));
#16909=DIRECTION('ref_axis',(1.,0.,0.));
#16910=DIRECTION('',(0.,0.,-1.));
#16911=DIRECTION('center_axis',(0.,0.,1.));
#16912=DIRECTION('ref_axis',(1.,0.,0.));
#16913=DIRECTION('center_axis',(0.,0.,1.));
#16914=DIRECTION('ref_axis',(1.,0.,0.));
#16915=DIRECTION('',(0.,0.,-1.));
#16916=DIRECTION('center_axis',(0.,0.,-1.));
#16917=DIRECTION('ref_axis',(1.,0.,0.));
#16918=DIRECTION('center_axis',(0.,0.,-1.));
#16919=DIRECTION('ref_axis',(1.,0.,0.));
#16920=DIRECTION('center_axis',(0.,0.,-1.));
#16921=DIRECTION('ref_axis',(1.,0.,0.));
#16922=DIRECTION('',(0.,0.,-1.));
#16923=DIRECTION('center_axis',(0.,0.,1.));
#16924=DIRECTION('ref_axis',(1.,0.,0.));
#16925=DIRECTION('center_axis',(0.,0.,-1.));
#16926=DIRECTION('ref_axis',(1.,0.,0.));
#16927=DIRECTION('center_axis',(0.,0.,-1.));
#16928=DIRECTION('ref_axis',(1.,0.,0.));
#16929=DIRECTION('',(0.,0.,-1.));
#16930=DIRECTION('center_axis',(0.,0.,1.));
#16931=DIRECTION('ref_axis',(1.,0.,0.));
#16932=DIRECTION('center_axis',(0.,0.,-1.));
#16933=DIRECTION('ref_axis',(1.,0.,0.));
#16934=DIRECTION('center_axis',(0.,0.,-1.));
#16935=DIRECTION('ref_axis',(1.,0.,0.));
#16936=DIRECTION('',(0.,0.,-1.));
#16937=DIRECTION('center_axis',(0.,0.,1.));
#16938=DIRECTION('ref_axis',(1.,0.,0.));
#16939=DIRECTION('center_axis',(0.,0.,-1.));
#16940=DIRECTION('ref_axis',(1.,0.,0.));
#16941=DIRECTION('center_axis',(0.,0.,-1.));
#16942=DIRECTION('ref_axis',(1.,0.,0.));
#16943=DIRECTION('',(0.,0.,-1.));
#16944=DIRECTION('center_axis',(0.,0.,1.));
#16945=DIRECTION('ref_axis',(1.,0.,0.));
#16946=DIRECTION('center_axis',(0.,0.,-1.));
#16947=DIRECTION('ref_axis',(1.,0.,0.));
#16948=DIRECTION('center_axis',(0.,0.,-1.));
#16949=DIRECTION('ref_axis',(1.,0.,0.));
#16950=DIRECTION('',(0.,0.,-1.));
#16951=DIRECTION('center_axis',(0.,0.,1.));
#16952=DIRECTION('ref_axis',(1.,0.,0.));
#16953=DIRECTION('center_axis',(0.,0.,-1.));
#16954=DIRECTION('ref_axis',(1.,0.,0.));
#16955=DIRECTION('center_axis',(0.,0.,-1.));
#16956=DIRECTION('ref_axis',(1.,0.,0.));
#16957=DIRECTION('',(0.,0.,-1.));
#16958=DIRECTION('center_axis',(0.,0.,1.));
#16959=DIRECTION('ref_axis',(1.,0.,0.));
#16960=DIRECTION('center_axis',(0.,1.,0.));
#16961=DIRECTION('ref_axis',(-1.,0.,0.));
#16962=DIRECTION('',(-1.,0.,0.));
#16963=DIRECTION('',(0.,0.,1.));
#16964=DIRECTION('',(-1.,0.,0.));
#16965=DIRECTION('center_axis',(1.,0.,0.));
#16966=DIRECTION('ref_axis',(0.,1.,0.));
#16967=DIRECTION('',(0.,1.,0.));
#16968=DIRECTION('',(0.,1.,0.));
#16969=DIRECTION('',(0.,0.,1.));
#16970=DIRECTION('center_axis',(0.,-1.,0.));
#16971=DIRECTION('ref_axis',(1.,0.,0.));
#16972=DIRECTION('',(1.,0.,0.));
#16973=DIRECTION('',(1.,0.,0.));
#16974=DIRECTION('center_axis',(0.,0.,1.));
#16975=DIRECTION('ref_axis',(1.,0.,0.));
#16976=DIRECTION('center_axis',(0.,0.,1.));
#16977=DIRECTION('ref_axis',(1.,0.,0.));
#16978=DIRECTION('center_axis',(0.,0.,1.));
#16979=DIRECTION('ref_axis',(1.,0.,0.));
#16980=DIRECTION('center_axis',(0.,0.,1.));
#16981=DIRECTION('ref_axis',(1.,0.,0.));
#16982=DIRECTION('center_axis',(0.,0.,1.));
#16983=DIRECTION('ref_axis',(1.,0.,0.));
#16984=DIRECTION('center_axis',(0.,0.,-1.));
#16985=DIRECTION('ref_axis',(1.,0.,0.));
#16986=DIRECTION('center_axis',(0.,0.,1.));
#16987=DIRECTION('ref_axis',(1.,0.,0.));
#16988=DIRECTION('',(0.,0.,-1.));
#16989=DIRECTION('center_axis',(0.,0.,1.));
#16990=DIRECTION('ref_axis',(1.,0.,0.));
#16991=DIRECTION('',(0.,0.,-1.));
#16992=DIRECTION('center_axis',(0.,0.,1.));
#16993=DIRECTION('ref_axis',(1.,0.,0.));
#16994=DIRECTION('center_axis',(0.,0.,1.));
#16995=DIRECTION('ref_axis',(1.,0.,0.));
#16996=DIRECTION('center_axis',(0.,0.,-1.));
#16997=DIRECTION('ref_axis',(1.,0.,0.));
#16998=DIRECTION('',(0.,0.,-1.));
#16999=DIRECTION('',(0.,0.,-1.));
#17000=DIRECTION('center_axis',(0.,0.,-1.));
#17001=DIRECTION('ref_axis',(1.,0.,0.));
#17002=DIRECTION('center_axis',(0.,0.,1.));
#17003=DIRECTION('ref_axis',(1.,0.,0.));
#17004=DIRECTION('center_axis',(0.,0.,1.));
#17005=DIRECTION('ref_axis',(1.,0.,0.));
#19951=CARTESIAN_POINT('',(0.,0.,0.));
#19952=CARTESIAN_POINT('Origin',(-46.,-3.,140.));
#19953=CARTESIAN_POINT('',(-49.9099188538711,-3.,80.));
#19954=CARTESIAN_POINT('',(-49.9099188538711,-3.,140.));
#19955=CARTESIAN_POINT('',(-49.9099188538711,-3.,60.));
#19956=CARTESIAN_POINT('',(-54.,-3.,80.));
#19957=CARTESIAN_POINT('',(-54.,-3.,80.));
#19958=CARTESIAN_POINT('',(-54.,-3.,140.));
#19959=CARTESIAN_POINT('',(-54.,-3.,140.));
#19960=CARTESIAN_POINT('',(-54.,-3.,140.));
#19961=CARTESIAN_POINT('Origin',(-50.,0.,140.));
#19962=CARTESIAN_POINT('',(-50.,-6.12323399573677E-15,140.));
#19963=CARTESIAN_POINT('Origin',(0.,0.,140.));
#19964=CARTESIAN_POINT('',(-54.,3.,140.));
#19965=CARTESIAN_POINT('',(-54.,3.,140.));
#19966=CARTESIAN_POINT('',(-49.9099188538711,3.,140.));
#19967=CARTESIAN_POINT('',(-46.,3.,140.));
#19968=CARTESIAN_POINT('Origin',(0.,0.,140.));
#19969=CARTESIAN_POINT('Origin',(-54.,3.,140.));
#19970=CARTESIAN_POINT('',(-49.9099188538711,3.,80.));
#19971=CARTESIAN_POINT('',(-49.9099188538711,3.,60.));
#19972=CARTESIAN_POINT('',(-54.,3.,80.));
#19973=CARTESIAN_POINT('',(-54.,3.,140.));
#19974=CARTESIAN_POINT('',(-46.,3.,80.));
#19975=CARTESIAN_POINT('Origin',(-54.,-3.,140.));
#19976=CARTESIAN_POINT('',(-54.,3.,80.));
#19977=CARTESIAN_POINT('Origin',(-50.,0.,80.));
#19978=CARTESIAN_POINT('',(-50.,-6.12323399573677E-15,80.));
#19979=CARTESIAN_POINT('Origin',(0.,0.,80.));
#19980=CARTESIAN_POINT('Origin',(0.,0.,80.));
#19981=CARTESIAN_POINT('Origin',(80.,0.,146.));
#19982=CARTESIAN_POINT('',(69.725,6.19873979128017,146.));
#19983=CARTESIAN_POINT('',(69.725,-6.19873979128017,146.));
#19984=CARTESIAN_POINT('Origin',(0.,0.,146.));
#19985=CARTESIAN_POINT('Origin',(80.,0.,146.));
#19986=CARTESIAN_POINT('Origin',(80.,0.,148.));
#19987=CARTESIAN_POINT('',(69.725,6.19873979128013,150.));
#19988=CARTESIAN_POINT('',(69.725,6.19873979128017,148.));
#19989=CARTESIAN_POINT('',(69.725,-6.19873979128013,150.));
#19990=CARTESIAN_POINT('Origin',(80.,0.,150.));
#19991=CARTESIAN_POINT('',(69.725,-6.19873979128017,148.));
#19992=CARTESIAN_POINT('Origin',(0.,0.,60.));
#19993=CARTESIAN_POINT('',(68.3739716558867,-15.,150.));
#19994=CARTESIAN_POINT('Origin',(0.,0.,150.));
#19995=CARTESIAN_POINT('',(68.3739716558867,-15.,160.));
#19996=CARTESIAN_POINT('',(68.3739716558867,-15.,60.));
#19997=CARTESIAN_POINT('',(-70.,-8.57252759403147E-15,160.));
#19998=CARTESIAN_POINT('Origin',(0.,0.,160.));
#19999=CARTESIAN_POINT('',(-70.,-8.57252759403147E-15,110.));
#20000=CARTESIAN_POINT('',(-70.,-8.57252759403147E-15,60.));
#20001=CARTESIAN_POINT('Origin',(0.,0.,110.));
#20002=CARTESIAN_POINT('',(68.3739716558867,15.,160.));
#20003=CARTESIAN_POINT('Origin',(0.,0.,160.));
#20004=CARTESIAN_POINT('',(68.3739716558867,15.,150.));
#20005=CARTESIAN_POINT('',(68.3739716558867,15.,60.));
#20006=CARTESIAN_POINT('Origin',(0.,0.,150.));
#20007=CARTESIAN_POINT('Origin',(80.,0.,155.));
#20008=CARTESIAN_POINT('',(72.,9.79717439317883E-16,160.));
#20009=CARTESIAN_POINT('Origin',(80.,0.,160.));
#20010=CARTESIAN_POINT('',(72.,9.79717439317883E-16,150.));
#20011=CARTESIAN_POINT('',(72.,9.79717439317883E-16,155.));
#20012=CARTESIAN_POINT('Origin',(80.,0.,150.));
#20013=CARTESIAN_POINT('Origin',(80.,0.,100.));
#20014=CARTESIAN_POINT('',(72.,9.79717439317883E-16,110.));
#20015=CARTESIAN_POINT('Origin',(80.,0.,110.));
#20016=CARTESIAN_POINT('',(72.,9.79717439317883E-16,90.));
#20017=CARTESIAN_POINT('',(72.,9.79717439317883E-16,100.));
#20018=CARTESIAN_POINT('Origin',(80.,0.,90.));
#20019=CARTESIAN_POINT('Origin',(60.,-60.,100.));
#20020=CARTESIAN_POINT('',(54.5,-60.,110.));
#20021=CARTESIAN_POINT('Origin',(60.,-60.,110.));
#20022=CARTESIAN_POINT('',(54.5,-60.,90.));
#20023=CARTESIAN_POINT('',(54.5,-60.,100.));
#20024=CARTESIAN_POINT('Origin',(60.,-60.,90.));
#20025=CARTESIAN_POINT('Origin',(-60.,-60.,100.));
#20026=CARTESIAN_POINT('',(-65.5,-60.,110.));
#20027=CARTESIAN_POINT('Origin',(-60.,-60.,110.));
#20028=CARTESIAN_POINT('',(-65.5,-60.,90.));
#20029=CARTESIAN_POINT('',(-65.5,-60.,100.));
#20030=CARTESIAN_POINT('Origin',(-60.,-60.,90.));
#20031=CARTESIAN_POINT('Origin',(-60.,60.,100.));
#20032=CARTESIAN_POINT('',(-65.5,60.,110.));
#20033=CARTESIAN_POINT('Origin',(-60.,60.,110.));
#20034=CARTESIAN_POINT('',(-65.5,60.,90.));
#20035=CARTESIAN_POINT('',(-65.5,60.,100.));
#20036=CARTESIAN_POINT('Origin',(-60.,60.,90.));
#20037=CARTESIAN_POINT('Origin',(60.,60.,100.));
#20038=CARTESIAN_POINT('',(54.5,60.,110.));
#20039=CARTESIAN_POINT('Origin',(60.,60.,110.));
#20040=CARTESIAN_POINT('',(54.5,60.,90.));
#20041=CARTESIAN_POINT('',(54.5,60.,100.));
#20042=CARTESIAN_POINT('Origin',(60.,60.,90.));
#20043=CARTESIAN_POINT('Origin',(100.,15.,150.));
#20044=CARTESIAN_POINT('',(100.,15.,160.));
#20045=CARTESIAN_POINT('',(100.,15.,160.));
#20046=CARTESIAN_POINT('',(100.,15.,150.));
#20047=CARTESIAN_POINT('',(100.,15.,150.));
#20048=CARTESIAN_POINT('',(100.,15.,150.));
#20049=CARTESIAN_POINT('Origin',(100.,-15.,150.));
#20050=CARTESIAN_POINT('',(100.,-15.,150.));
#20051=CARTESIAN_POINT('',(100.,-15.,150.));
#20052=CARTESIAN_POINT('',(100.,-15.,160.));
#20053=CARTESIAN_POINT('',(100.,-15.,160.));
#20054=CARTESIAN_POINT('',(100.,-15.,150.));
#20055=CARTESIAN_POINT('Origin',(50.,-15.,150.));
#20056=CARTESIAN_POINT('',(50.,-15.,150.));
#20057=CARTESIAN_POINT('',(50.,-15.,160.));
#20058=CARTESIAN_POINT('Origin',(75.,0.,150.));
#20059=CARTESIAN_POINT('Origin',(0.,0.,110.));
#20060=CARTESIAN_POINT('',(-100.,-1.22464679914735E-14,110.));
#20061=CARTESIAN_POINT('Origin',(0.,0.,110.));
#20062=CARTESIAN_POINT('Origin',(0.,0.,90.));
#20063=CARTESIAN_POINT('',(-100.,-1.22464679914735E-14,90.));
#20064=CARTESIAN_POINT('Origin',(0.,0.,90.));
#20065=CARTESIAN_POINT('',(-70.,8.57252759403147E-15,90.));
#20066=CARTESIAN_POINT('Origin',(0.,0.,90.));
#20067=CARTESIAN_POINT('Origin',(0.,0.,90.));
#20068=CARTESIAN_POINT('',(-100.,-1.22464679914735E-14,90.));
#20069=CARTESIAN_POINT('Origin',(0.,0.,60.));
#20070=CARTESIAN_POINT('',(-70.,-8.57252759403147E-15,60.));
#20071=CARTESIAN_POINT('',(-70.,-8.57252759403147E-15,60.));
#20072=CARTESIAN_POINT('Origin',(0.,0.,60.));
#20073=CARTESIAN_POINT('Origin',(0.,0.,60.));
#20074=CARTESIAN_POINT('',(-50.,-6.12323399573677E-15,160.));
#20075=CARTESIAN_POINT('Origin',(0.,0.,160.));
#20076=CARTESIAN_POINT('',(-50.,-6.12323399573677E-15,60.));
#20077=CARTESIAN_POINT('',(-50.,-6.12323399573677E-15,60.));
#20078=CARTESIAN_POINT('',(-50.,-6.12323399573677E-15,60.));
#20079=CARTESIAN_POINT('Origin',(0.,0.,60.));
#20080=CARTESIAN_POINT('Origin',(0.,0.,160.));
#20081=CARTESIAN_POINT('Origin',(0.,0.,60.));
#63860=UNCERTAINTY_MEASURE_WITH_UNIT(LENGTH_MEASURE(0.01),#63899,
'DISTANCE_ACCURACY_VALUE',
'Maximum model space distance between geometric entities at asserted c
onnectivities');
#63878=UNCERTAINTY_MEASURE_WITH_UNIT(LENGTH_MEASURE(0.01),#63899,
'DISTANCE_ACCURACY_VALUE',
'Maximum model space distance between geometric entities at asserted c
onnectivities');
#63880=(
GEOMETRIC_REPRESENTATION_CONTEXT(3)
GLOBAL_UNCERTAINTY_ASSIGNED_CONTEXT((#63860))
GLOBAL_UNIT_ASSIGNED_CONTEXT((#63899,#63901,#63902))
REPRESENTATION_CONTEXT('','3D')
);
#63898=(
GEOMETRIC_REPRESENTATION_CONTEXT(3)
GLOBAL_UNCERTAINTY_ASSIGNED_CONTEXT((#63878))
GLOBAL_UNIT_ASSIGNED_CONTEXT((#63899,#63901,#63902))
REPRESENTATION_CONTEXT('','3D')
);
#63899=(
LENGTH_UNIT()
NAMED_UNIT(*)
SI_UNIT(.MILLI.,.METRE.)
);
#63901=(
NAMED_UNIT(*)
PLANE_ANGLE_UNIT()
SI_UNIT($,.RADIAN.)
);
#63902=(
NAMED_UNIT(*)
SI_UNIT($,.STERADIAN.)
SOLID_ANGLE_UNIT()
);
#63904=SHAPE_DEFINITION_REPRESENTATION(#63923,#63995);
#63923=PRODUCT_DEFINITION_SHAPE('',$,#64015);
#63995=SHAPE_REPRESENTATION('',(#15696),#63880);
#64013=PRODUCT_DEFINITION_CONTEXT('part definition',#64072,'design');
#64015=PRODUCT_DEFINITION('Guide housing','Guide housing',#64034,#64013);
#64034=PRODUCT_DEFINITION_FORMATION('',$,#64075);
#64072=APPLICATION_CONTEXT(
'Core Data for Automotive Mechanical Design Process');
#64073=PRODUCT_CONTEXT('part definition',#64072,'mechanical');
#64075=PRODUCT('Guide housing','Guide housing',$,(#64073));
#64094=PRESENTATION_STYLE_ASSIGNMENT((#64107));
#64107=SURFACE_STYLE_USAGE(.BOTH.,#64120);
#64120=SURFACE_SIDE_STYLE('',(#64133));
#64133=SURFACE_STYLE_FILL_AREA(#64146);
#64146=FILL_AREA_STYLE('Dark blue',(#64159));
#64159=FILL_AREA_STYLE_COLOUR('Dark blue',#64172);
#64172=COLOUR_RGB('Dark blue',0.0901960784313725,0.270588235294118,0.513725490196078);
ENDSEC;
END-ISO-10303-21;
